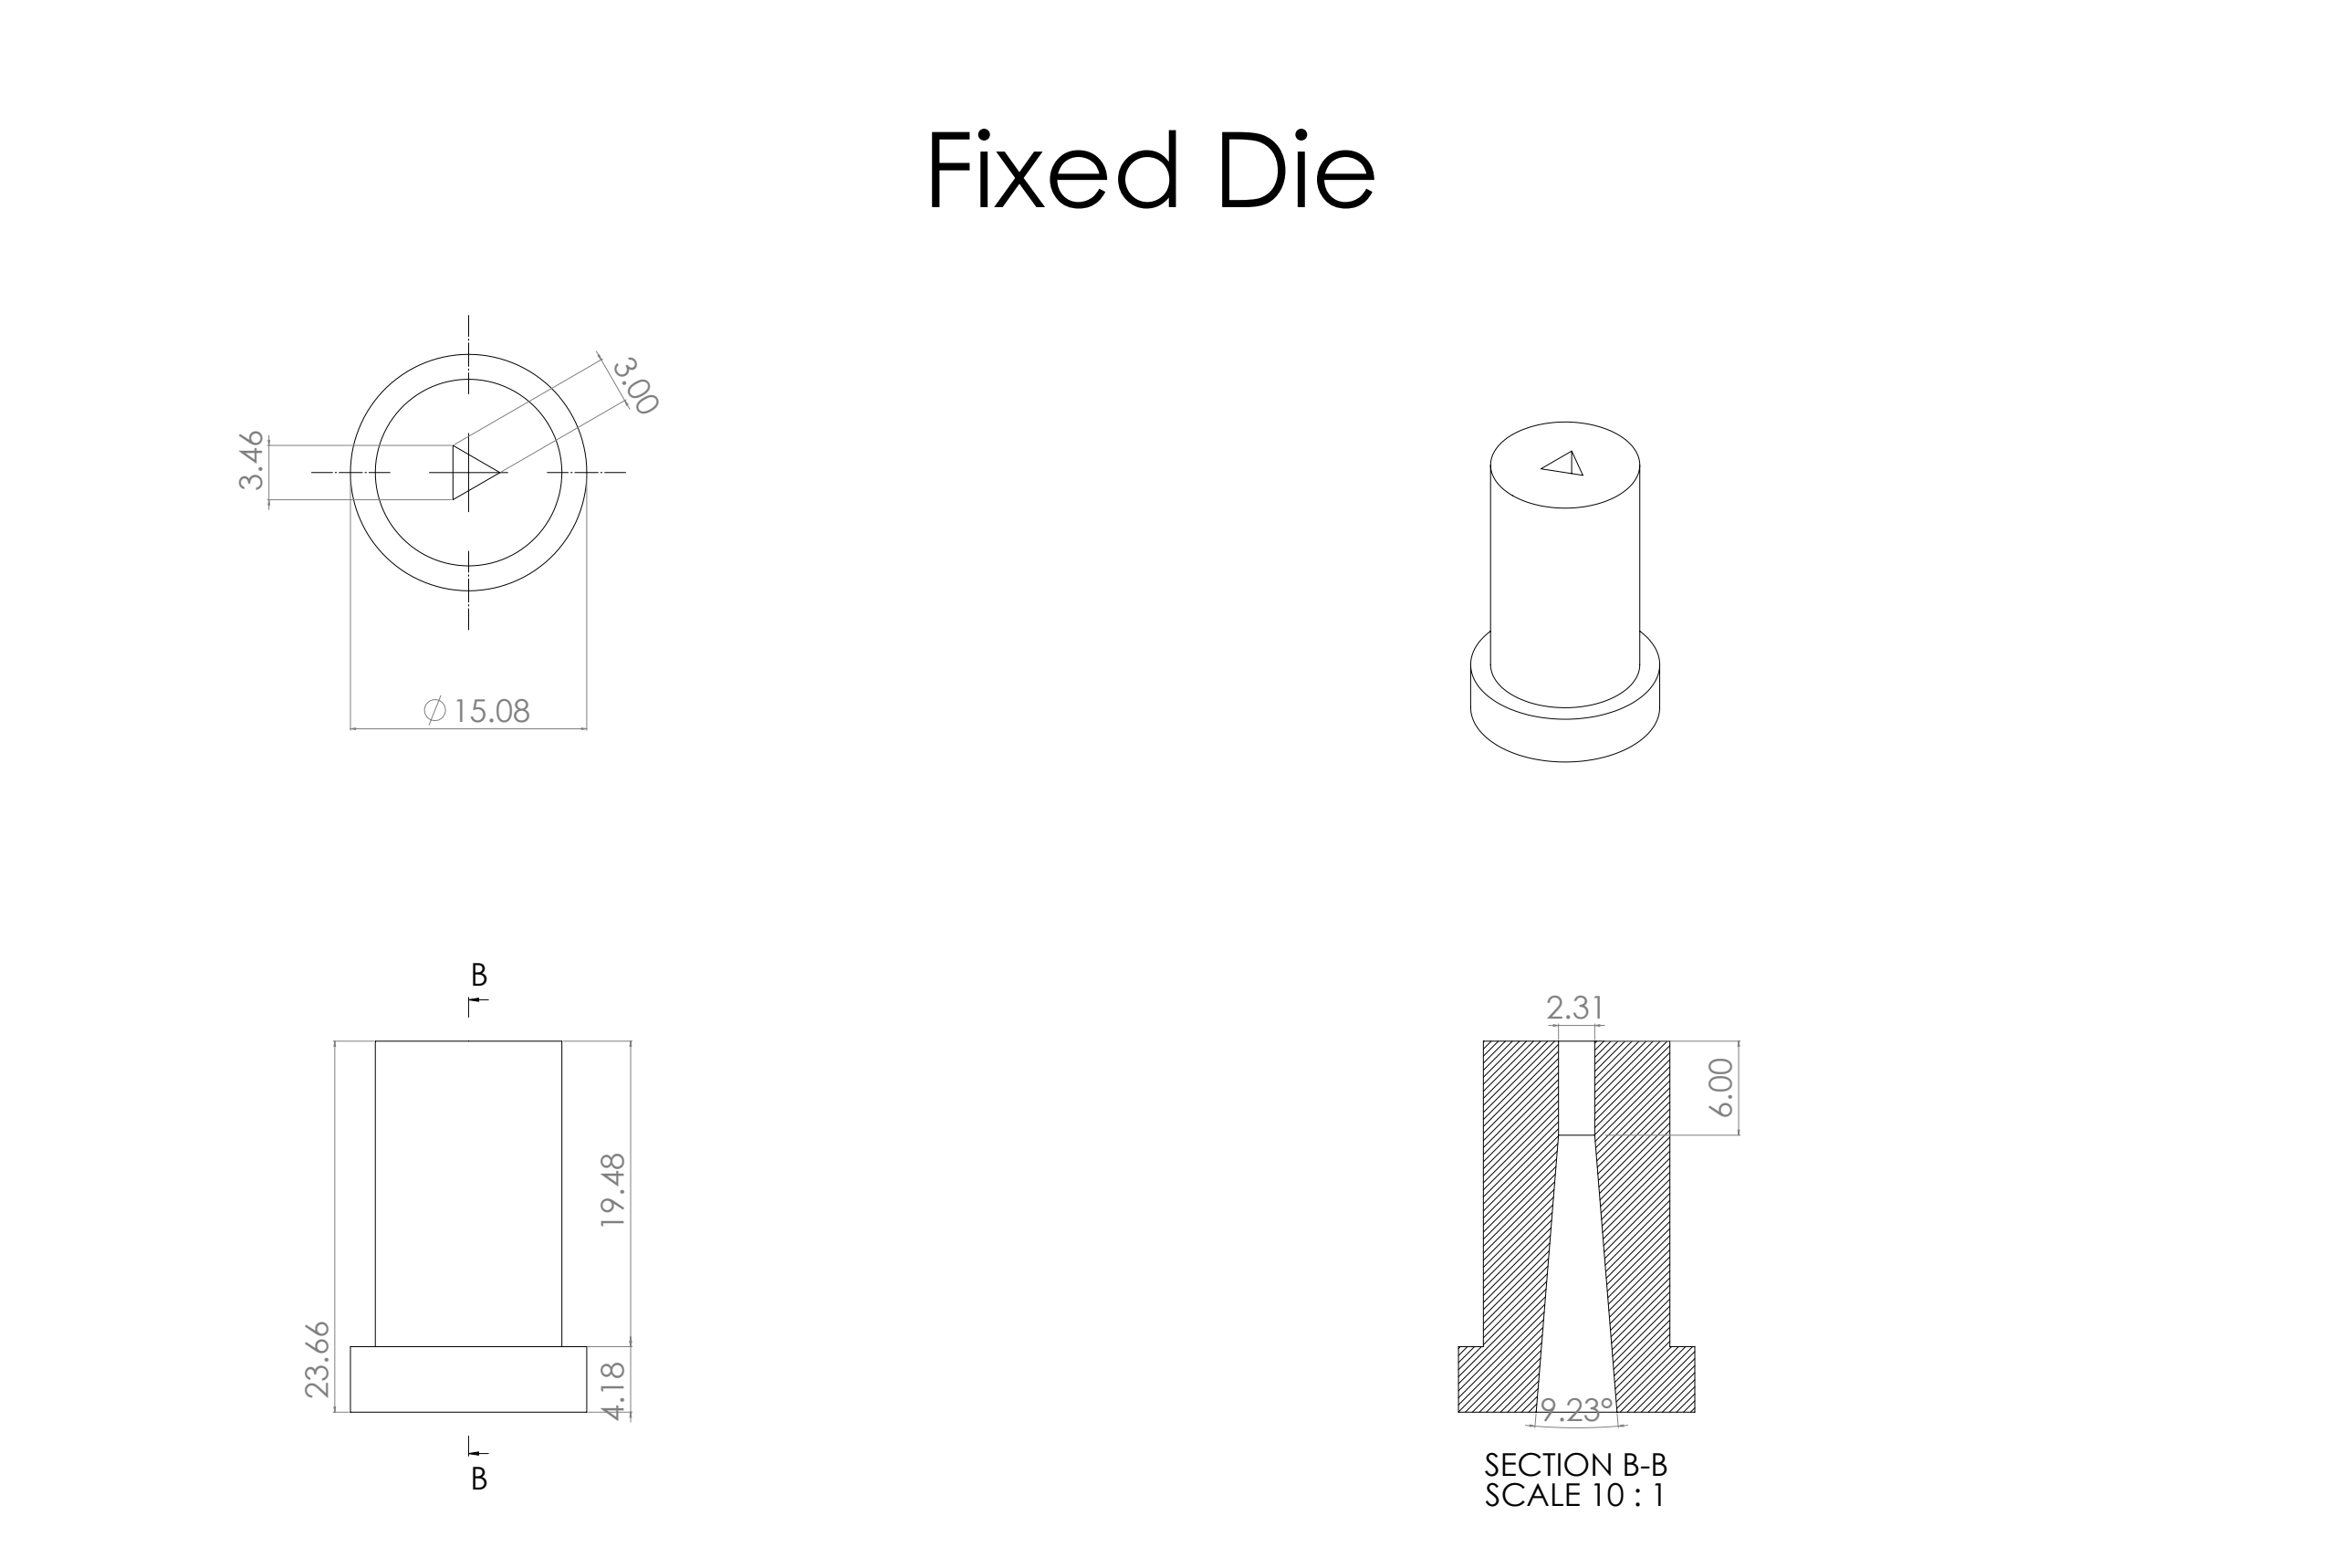
ISO-10303-21;
HEADER;
FILE_DESCRIPTION (('STEP AP214'),
    '1' );
FILE_NAME ('Fixed Die.step',
    '2026-10-24T22:54:28',
    ( '' ),
    ( '' ),
    'SwSTEP 2.0',
    'SolidWorks 2025',
    '' );
FILE_SCHEMA (( 'AUTOMOTIVE_DESIGN' ));
ENDSEC;

DATA;
#207=CARTESIAN_POINT ( 'NONE',  ( -71.92837670882106238, -36.87473357531881391, 0.000000000000000000 ) ) ;
#224=DIRECTION ( 'NONE',  ( 0.8660254037844378194, 0.000000000000000000, -0.5000000000000015543 ) ) ;
#393=VERTEX_POINT ( 'NONE', #4566 ) ;
#434=PLANE ( 'NONE',  #17404 ) ;
#625=EDGE_LOOP ( 'NONE', ( #4883, #27978 ) ) ;
#665=LINE ( 'NONE', #13201, #39699 ) ;
#902=LINE ( 'NONE', #25603, #35773 ) ;
#1067=( LENGTH_UNIT ( ) NAMED_UNIT ( * ) SI_UNIT ( .MILLI., .METRE. ) );
#1090=CARTESIAN_POINT ( 'NONE',  ( -70.92837670882107659, -56.35932253828836025, -7.538952224936807056 ) ) ;
#1093=EDGE_LOOP ( 'NONE', ( #23116, #22958, #9931 ) ) ;
#1109=EDGE_LOOP ( 'NONE', ( #22255, #22599 ) ) ;
#1161=EDGE_CURVE ( 'NONE', #12672, #5311, #17051, .T. ) ;
#1597=EDGE_CURVE ( 'NONE', #40141, #14437, #22702, .T. ) ;
#1683=CARTESIAN_POINT ( 'NONE',  ( -71.89960098016555889, -42.46322148352267334, 1.682209783512720325 ) ) ;
#1749=CARTESIAN_POINT ( 'NONE',  ( -70.92837670882107659, -36.87473357531881391, 5.950000000000010836 ) ) ;
#2203=DIRECTION ( 'NONE',  ( 0.000000000000000000, 1.000000000000000000, 0.000000000000000000 ) ) ;
#2209=DIRECTION ( 'NONE',  ( 0.000000000000000000, 0.000000000000000000, 1.000000000000000000 ) ) ;
#2300=AXIS2_PLACEMENT_3D ( 'NONE', #39101, #26169, #4151 ) ;
#2364=LINE ( 'NONE', #33652, #10169 ) ;
#2727=CARTESIAN_POINT ( 'NONE',  ( -64.15669616364040451, -60.53509472482660669, 1.328953532546354177 ) ) ;
#2806=DIRECTION ( 'NONE',  ( 0.000000000000000000, 1.000000000000000000, 0.000000000000000000 ) ) ;
#2845=PRODUCT_DEFINITION_CONTEXT ( 'detailed design', #4008, 'design' ) ;
#2876=PLANE ( 'NONE',  #36603 ) ;
#2926=DIRECTION ( 'NONE',  ( 0.000000000000000000, 0.000000000000000000, -1.000000000000000000 ) ) ;
#2936=VECTOR ( 'NONE', #14406, 1000.000000000000000 ) ;
#2937=VERTEX_POINT ( 'NONE', #1749 ) ;
#3000=CIRCLE ( 'NONE', #2300, 7.538952224936807056 ) ;
#3131=ORIENTED_EDGE ( 'NONE', *, *, #5528, .T. ) ;
#3396=DIRECTION ( 'NONE',  ( -0.000000000000000000, -1.000000000000000000, -0.000000000000000000 ) ) ;
#3415=LINE ( 'NONE', #15927, #25846 ) ;
#3420=FACE_OUTER_BOUND ( 'NONE', #15790, .T. ) ;
#3469=CARTESIAN_POINT ( 'NONE',  ( -70.92837670882107659, -56.35932253828836025, 0.000000000000000000 ) ) ;
#3553=DIRECTION ( 'NONE',  ( 1.000000000000000000, 0.000000000000000000, 0.000000000000000000 ) ) ;
#3613=EDGE_LOOP ( 'NONE', ( #15107, #25975, #24061, #17576 ) ) ;
#3750=( GEOMETRIC_REPRESENTATION_CONTEXT ( 3 ) GLOBAL_UNCERTAINTY_ASSIGNED_CONTEXT ( ( #25460 ) ) GLOBAL_UNIT_ASSIGNED_CONTEXT ( ( #39616, #24183, #17995 ) ) REPRESENTATION_CONTEXT ( 'NONE', 'WORKASPACE' ) );
#3827=CARTESIAN_POINT ( 'NONE',  ( -70.92837670882107659, -36.87473357531881391, 0.000000000000000000 ) ) ;
#3963=CARTESIAN_POINT ( 'NONE',  ( -71.92837670882106238, -42.87473357531881391, -1.732050807568860318 ) ) ;
#4008=APPLICATION_CONTEXT ( 'automotive_design' ) ;
#4151=DIRECTION ( 'NONE',  ( 0.000000000000000000, 0.000000000000000000, -1.000000000000000000 ) ) ;
#4259=DIRECTION ( 'NONE',  ( 0.000000000000000000, 0.000000000000000000, -1.000000000000000000 ) ) ;
#4566=CARTESIAN_POINT ( 'NONE',  ( -70.92837670882107659, -60.53509472482660669, 7.538952224936807056 ) ) ;
#4749=CARTESIAN_POINT ( 'NONE',  ( -66.45851120290885206, -60.53509472482660669, -7.806255641895631925E-15 ) ) ;
#4780=VERTEX_POINT ( 'NONE', #9078 ) ;
#4883=ORIENTED_EDGE ( 'NONE', *, *, #31531, .F. ) ;
#5208=VERTEX_POINT ( 'NONE', #4749 ) ;
#5311=VERTEX_POINT ( 'NONE', #14408 ) ;
#5366=ORIENTED_EDGE ( 'NONE', *, *, #5820, .T. ) ;
#5526=CARTESIAN_POINT ( 'NONE',  ( -71.92837670882106238, -42.87473357531881391, -1.732050807568860318 ) ) ;
#5528=EDGE_CURVE ( 'NONE', #24744, #4780, #6786, .T. ) ;
#5754=VERTEX_POINT ( 'NONE', #7183 ) ;
#5820=EDGE_CURVE ( 'NONE', #5754, #35842, #23779, .T. ) ;
#5942=CARTESIAN_POINT ( 'NONE',  ( -70.42837670882107659, -36.87473357531881391, -0.8660254037844368202 ) ) ;
#6122=AXIS2_PLACEMENT_3D ( 'NONE', #20569, #33156, #7623 ) ;
#6322=ORIENTED_EDGE ( 'NONE', *, *, #1161, .F. ) ;
#6624=CARTESIAN_POINT ( 'NONE',  ( -71.92837670882106238, -36.87473357531881391, -1.732050807568860318 ) ) ;
#6666=EDGE_CURVE ( 'NONE', #2937, #18869, #36703, .T. ) ;
#6714=AXIS2_PLACEMENT_3D ( 'NONE', #38265, #38664, #32717 ) ;
#6786=LINE ( 'NONE', #207, #20487 ) ;
#7021=FACE_OUTER_BOUND ( 'NONE', #11884, .T. ) ;
#7183=CARTESIAN_POINT ( 'NONE',  ( -70.92837670882107659, -56.35932253828836025, 7.538952224936807056 ) ) ;
#7203=CARTESIAN_POINT ( 'NONE',  ( -70.92837670882107659, -60.53509472482660669, -7.538952224936807056 ) ) ;
#7316=PRODUCT_CONTEXT ( 'NONE', #8952, 'mechanical' ) ;
#7549=DIRECTION ( 'NONE',  ( 0.000000000000000000, 0.000000000000000000, -1.000000000000000000 ) ) ;
#7594=DIRECTION ( 'NONE',  ( 0.8660254037844378194, 0.000000000000000000, -0.5000000000000015543 ) ) ;
#7623=DIRECTION ( 'NONE',  ( 0.8660254037844378194, 0.000000000000000000, -0.5000000000000015543 ) ) ;
#7919=SHAPE_DEFINITION_REPRESENTATION ( #12565, #32460 ) ;
#7949=EDGE_CURVE ( 'NONE', #22149, #393, #24947, .T. ) ;
#7985=CYLINDRICAL_SURFACE ( 'NONE', #23972, 5.950000000000010836 ) ;
#8004=DIRECTION ( 'NONE',  ( -0.000000000000000000, -1.000000000000000000, -0.000000000000000000 ) ) ;
#8100=ORIENTED_EDGE ( 'NONE', *, *, #8860, .T. ) ;
#8103=DIRECTION ( 'NONE',  ( -0.000000000000000000, 1.000000000000000000, -0.000000000000000000 ) ) ;
#8110=ORIENTED_EDGE ( 'NONE', *, *, #25965, .T. ) ;
#8132=CARTESIAN_POINT ( 'NONE',  ( -71.92837670882106238, -42.87473357531881391, 1.732050807568877637 ) ) ;
#8190=AXIS2_PLACEMENT_3D ( 'NONE', #18545, #27616, #27209 ) ;
#8239=PRODUCT ( 'Fixed Die', 'Fixed Die', '', ( #7316 ) ) ;
#8244=LINE ( 'NONE', #2727, #8578 ) ;
#8344=DIRECTION ( 'NONE',  ( 0.000000000000000000, -0.000000000000000000, 1.000000000000000000 ) ) ;
#8361=EDGE_LOOP ( 'NONE', ( #33245, #39618, #23431, #8597 ) ) ;
#8539=CARTESIAN_POINT ( 'NONE',  ( -71.92837670882106238, -42.87473357531881391, 1.732050807568877637 ) ) ;
#8569=UNCERTAINTY_MEASURE_WITH_UNIT (LENGTH_MEASURE( 1.000000000000000082E-05 ), #1067, 'distance_accuracy_value', 'NONE');
#8578=VECTOR ( 'NONE', #15250, 1000.000000000000114 ) ;
#8597=ORIENTED_EDGE ( 'NONE', *, *, #24404, .F. ) ;
#8860=EDGE_CURVE ( 'NONE', #2937, #5311, #17859, .T. ) ;
#8948=DIRECTION ( 'NONE',  ( 0.000000000000000000, 0.000000000000000000, -1.000000000000000000 ) ) ;
#8952=APPLICATION_CONTEXT ( 'automotive_design' ) ;
#8971=AXIS2_PLACEMENT_3D ( 'NONE', #30800, #2806, #27681 ) ;
#9068=CARTESIAN_POINT ( 'NONE',  ( -68.92837670882107659, -42.87473357531881391, 0.000000000000000000 ) ) ;
#9078=CARTESIAN_POINT ( 'NONE',  ( -71.92837670882106238, -36.87473357531881391, 1.732050807568877637 ) ) ;
#9085=DIRECTION ( 'NONE',  ( -0.000000000000000000, -1.000000000000000000, -0.000000000000000000 ) ) ;
#9329=EDGE_LOOP ( 'NONE', ( #30157, #30991, #26917 ) ) ;
#9485=DIRECTION ( 'NONE',  ( 0.000000000000000000, 0.000000000000000000, 1.000000000000000000 ) ) ;
#9529=CIRCLE ( 'NONE', #39079, 5.950000000000010836 ) ;
#9571=FACE_BOUND ( 'NONE', #1093, .T. ) ;
#9887=FACE_OUTER_BOUND ( 'NONE', #33067, .T. ) ;
#9931=ORIENTED_EDGE ( 'NONE', *, *, #10183, .F. ) ;
#10141=DIRECTION ( 'NONE',  ( 0.06925283225918045515, 0.9903616414705930238, 0.1199494240409451351 ) ) ;
#10152=DIRECTION ( 'NONE',  ( 0.000000000000000000, 0.000000000000000000, -1.000000000000000000 ) ) ;
#10169=VECTOR ( 'NONE', #15091, 1000.000000000000114 ) ;
#10183=EDGE_CURVE ( 'NONE', #21412, #5208, #8244, .T. ) ;
#10234=DIRECTION ( 'NONE',  ( -0.000000000000000000, -1.000000000000000000, -0.000000000000000000 ) ) ;
#11063=ORIENTED_EDGE ( 'NONE', *, *, #36631, .T. ) ;
#11143=AXIS2_PLACEMENT_3D ( 'NONE', #3469, #22995, #4259 ) ;
#11295=PLANE ( 'NONE',  #6122 ) ;
#11801=ORIENTED_EDGE ( 'NONE', *, *, #1597, .F. ) ;
#11884=EDGE_LOOP ( 'NONE', ( #26290, #20183, #23152, #11801 ) ) ;
#12137=ORIENTED_EDGE ( 'NONE', *, *, #12369, .F. ) ;
#12246=DIRECTION ( 'NONE',  ( 0.000000000000000000, -1.000000000000000000, -0.000000000000000000 ) ) ;
#12369=EDGE_CURVE ( 'NONE', #28633, #31670, #2364, .T. ) ;
#12447=AXIS2_PLACEMENT_3D ( 'NONE', #33798, #24304, #2926 ) ;
#12478=VECTOR ( 'NONE', #26746, 1000.000000000000000 ) ;
#12565=PRODUCT_DEFINITION_SHAPE ( 'NONE', 'NONE',  #27315 ) ;
#12595=EDGE_CURVE ( 'NONE', #18869, #2937, #9529, .T. ) ;
#12657=PLANE ( 'NONE',  #30715 ) ;
#12672=VERTEX_POINT ( 'NONE', #39135 ) ;
#12682=SHAPE_REPRESENTATION_RELATIONSHIP ( 'NONE' , 'NONE' ,  #32460, #31867 ) ;
#13056=ADVANCED_FACE ( 'NONE', ( #30915 ), #434, .F. ) ;
#13093=( NAMED_UNIT ( * ) PLANE_ANGLE_UNIT ( ) SI_UNIT ( $, .RADIAN. ) );
#13201=CARTESIAN_POINT ( 'NONE',  ( -64.15669616364041872, -60.53509472482660669, -1.328953532546369276 ) ) ;
#13407=FACE_BOUND ( 'NONE', #1109, .T. ) ;
#13587=EDGE_CURVE ( 'NONE', #15847, #24744, #21594, .T. ) ;
#14273=EDGE_LOOP ( 'NONE', ( #15186, #5366, #11063, #14688 ) ) ;
#14366=DIRECTION ( 'NONE',  ( -0.000000000000000000, -1.000000000000000000, -0.000000000000000000 ) ) ;
#14406=DIRECTION ( 'NONE',  ( 0.000000000000000000, 0.000000000000000000, -1.000000000000000000 ) ) ;
#14408=CARTESIAN_POINT ( 'NONE',  ( -70.92837670882107659, -56.35932253828836025, 5.950000000000010836 ) ) ;
#14437=VERTEX_POINT ( 'NONE', #8132 ) ;
#14588=EDGE_CURVE ( 'NONE', #5754, #393, #18017, .T. ) ;
#14637=FACE_OUTER_BOUND ( 'NONE', #8361, .T. ) ;
#14662=DIRECTION ( 'NONE',  ( 0.000000000000000000, 0.000000000000000000, -1.000000000000000000 ) ) ;
#14688=ORIENTED_EDGE ( 'NONE', *, *, #22477, .F. ) ;
#14692=CARTESIAN_POINT ( 'NONE',  ( -68.92837670882107659, -42.87473357531881391, 0.000000000000000000 ) ) ;
#14716=DIRECTION ( 'NONE',  ( -0.000000000000000000, -1.000000000000000000, -0.000000000000000000 ) ) ;
#14961=CARTESIAN_POINT ( 'NONE',  ( -73.16330946177717465, -60.53509472482661380, 3.871017079619767376 ) ) ;
#14986=ORIENTED_EDGE ( 'NONE', *, *, #28741, .T. ) ;
#15091=DIRECTION ( 'NONE',  ( -0.8660254037844399289, 0.000000000000000000, -0.4999999999999977240 ) ) ;
#15107=ORIENTED_EDGE ( 'NONE', *, *, #30928, .T. ) ;
#15126=PLANE ( 'NONE',  #8971 ) ;
#15186=ORIENTED_EDGE ( 'NONE', *, *, #14588, .F. ) ;
#15223=ORIENTED_EDGE ( 'NONE', *, *, #13587, .T. ) ;
#15250=DIRECTION ( 'NONE',  ( 0.8660254037844399289, 0.000000000000000000, 0.4999999999999976685 ) ) ;
#15444=ORIENTED_EDGE ( 'NONE', *, *, #12595, .F. ) ;
#15510=VECTOR ( 'NONE', #27833, 1000.000000000000114 ) ;
#15608=DIRECTION ( 'NONE',  ( 0.000000000000000000, 0.000000000000000000, 1.000000000000000000 ) ) ;
#15636=ADVANCED_FACE ( 'NONE', ( #38836 ), #35775, .T. ) ;
#15670=ADVANCED_FACE ( 'NONE', ( #23604, #33503 ), #18022, .T. ) ;
#15737=ORIENTED_EDGE ( 'NONE', *, *, #22477, .T. ) ;
#15790=EDGE_LOOP ( 'NONE', ( #32669, #22324, #37632, #26866 ) ) ;
#15832=ORIENTED_EDGE ( 'NONE', *, *, #32968, .T. ) ;
#15847=VERTEX_POINT ( 'NONE', #40074 ) ;
#15861=DIRECTION ( 'NONE',  ( -0.8660254037844399289, 0.000000000000000000, -0.4999999999999977240 ) ) ;
#15927=CARTESIAN_POINT ( 'NONE',  ( -71.92837670882106238, -42.87473357531881391, 1.732050807568877637 ) ) ;
#16115=CARTESIAN_POINT ( 'NONE',  ( -70.92837670882107659, -36.87473357531881391, 0.000000000000000000 ) ) ;
#16212=MECHANICAL_DESIGN_GEOMETRIC_PRESENTATION_REPRESENTATION('',(#39862),#3750);
#16213=VECTOR ( 'NONE', #30275, 1000.000000000000000 ) ;
#16974=LINE ( 'NONE', #14692, #28770 ) ;
#17017=ORIENTED_EDGE ( 'NONE', *, *, #12595, .T. ) ;
#17051=CIRCLE ( 'NONE', #11143, 5.950000000000010836 ) ;
#17091=CARTESIAN_POINT ( 'NONE',  ( -70.92837670882107659, -60.53509472482660669, -7.538952224936807056 ) ) ;
#17193=CARTESIAN_POINT ( 'NONE',  ( -71.92837670882106238, -42.87473357531881391, -1.732050807568860318 ) ) ;
#17300=AXIS2_PLACEMENT_3D ( 'NONE', #29110, #31800, #10152 ) ;
#17386=DIRECTION ( 'NONE',  ( -0.000000000000000000, 1.000000000000000000, -0.000000000000000000 ) ) ;
#17404=AXIS2_PLACEMENT_3D ( 'NONE', #37665, #18954, #224 ) ;
#17484=LINE ( 'NONE', #17091, #16213 ) ;
#17576=ORIENTED_EDGE ( 'NONE', *, *, #31764, .T. ) ;
#17612=CARTESIAN_POINT ( 'NONE',  ( -71.92837670882106238, -42.87473357531881391, -1.732050807568860318 ) ) ;
#17763=CARTESIAN_POINT ( 'NONE',  ( -73.16330946177717465, -60.53509472482659959, -3.871017079619738510 ) ) ;
#17820=LINE ( 'NONE', #17612, #26678 ) ;
#17859=LINE ( 'NONE', #30440, #12478 ) ;
#17995=( NAMED_UNIT ( * ) SI_UNIT ( $, .STERADIAN. ) SOLID_ANGLE_UNIT ( ) );
#18017=LINE ( 'NONE', #36559, #24725 ) ;
#18022=PLANE ( 'NONE',  #20626 ) ;
#18066=VECTOR ( 'NONE', #31067, 1000.000000000000114 ) ;
#18376=DIRECTION ( 'NONE',  ( -0.000000000000000000, 1.000000000000000000, -0.000000000000000000 ) ) ;
#18545=CARTESIAN_POINT ( 'NONE',  ( -68.92837670882107659, -42.87473357531881391, 0.000000000000000000 ) ) ;
#18660=AXIS2_PLACEMENT_3D ( 'NONE', #28786, #10234, #7549 ) ;
#18787=LINE ( 'NONE', #31365, #39256 ) ;
#18869=VERTEX_POINT ( 'NONE', #19058 ) ;
#18954=DIRECTION ( 'NONE',  ( 0.5000000000000015543, 0.000000000000000000, 0.8660254037844378194 ) ) ;
#19058=CARTESIAN_POINT ( 'NONE',  ( -70.92837670882107659, -36.87473357531881391, -5.950000000000010836 ) ) ;
#19589=PLANE ( 'NONE',  #33092 ) ;
#19592=VECTOR ( 'NONE', #17386, 1000.000000000000000 ) ;
#19700=LINE ( 'NONE', #8539, #19592 ) ;
#20177=DIRECTION ( 'NONE',  ( -0.9975640502598243087, 0.06975647374412531632, 0.000000000000000000 ) ) ;
#20183=ORIENTED_EDGE ( 'NONE', *, *, #24404, .T. ) ;
#20210=ADVANCED_FACE ( 'NONE', ( #36707 ), #20645, .T. ) ;
#20341=CARTESIAN_POINT ( 'NONE',  ( -70.42837670882107659, -36.87473357531881391, 0.8660254037844411501 ) ) ;
#20487=VECTOR ( 'NONE', #22033, 1000.000000000000000 ) ;
#20541=CARTESIAN_POINT ( 'NONE',  ( -70.92837670882107659, -60.53509472482660669, 0.000000000000000000 ) ) ;
#20569=CARTESIAN_POINT ( 'NONE',  ( -71.92837670882106238, -42.87473357531881391, 1.732050807568877637 ) ) ;
#20576=ORIENTED_EDGE ( 'NONE', *, *, #25965, .F. ) ;
#20617=ADVANCED_FACE ( 'NONE', ( #39074 ), #7985, .T. ) ;
#20626=AXIS2_PLACEMENT_3D ( 'NONE', #36168, #2203, #8344 ) ;
#20645=CYLINDRICAL_SURFACE ( 'NONE', #34514, 7.538952224936807056 ) ;
#20898=CIRCLE ( 'NONE', #35390, 7.538952224936807056 ) ;
#21412=VERTEX_POINT ( 'NONE', #17763 ) ;
#21594=LINE ( 'NONE', #5942, #18066 ) ;
#21733=FACE_OUTER_BOUND ( 'NONE', #32261, .T. ) ;
#21889=ORIENTED_EDGE ( 'NONE', *, *, #1597, .T. ) ;
#21909=ADVANCED_FACE ( 'NONE', ( #9887 ), #37271, .F. ) ;
#22033=DIRECTION ( 'NONE',  ( 0.000000000000000000, -0.000000000000000000, 1.000000000000000000 ) ) ;
#22075=LINE ( 'NONE', #25149, #40308 ) ;
#22128=ORIENTED_EDGE ( 'NONE', *, *, #7949, .T. ) ;
#22149=VERTEX_POINT ( 'NONE', #7203 ) ;
#22255=ORIENTED_EDGE ( 'NONE', *, *, #1161, .T. ) ;
#22276=ADVANCED_FACE ( 'NONE', ( #14637 ), #34238, .F. ) ;
#22324=ORIENTED_EDGE ( 'NONE', *, *, #14588, .T. ) ;
#22400=DIRECTION ( 'NONE',  ( 0.000000000000000000, 0.000000000000000000, -1.000000000000000000 ) ) ;
#22477=EDGE_CURVE ( 'NONE', #393, #22149, #3000, .T. ) ;
#22599=ORIENTED_EDGE ( 'NONE', *, *, #27281, .T. ) ;
#22702=LINE ( 'NONE', #1683, #22993 ) ;
#22958=ORIENTED_EDGE ( 'NONE', *, *, #32968, .F. ) ;
#22993=VECTOR ( 'NONE', #33172, 999.9999999999998863 ) ;
#22995=DIRECTION ( 'NONE',  ( -0.000000000000000000, -1.000000000000000000, -0.000000000000000000 ) ) ;
#23088=DIRECTION ( 'NONE',  ( -0.8660254037844377084, 0.000000000000000000, 0.5000000000000015543 ) ) ;
#23116=ORIENTED_EDGE ( 'NONE', *, *, #23514, .F. ) ;
#23144=DIRECTION ( 'NONE',  ( -0.000000000000000000, -1.000000000000000000, -0.000000000000000000 ) ) ;
#23152=ORIENTED_EDGE ( 'NONE', *, *, #35047, .T. ) ;
#23167=CIRCLE ( 'NONE', #32379, 5.950000000000010836 ) ;
#23431=ORIENTED_EDGE ( 'NONE', *, *, #12369, .T. ) ;
#23514=EDGE_CURVE ( 'NONE', #40141, #21412, #33163, .T. ) ;
#23604=FACE_BOUND ( 'NONE', #9329, .T. ) ;
#23626=ORIENTED_EDGE ( 'NONE', *, *, #38478, .T. ) ;
#23779=CIRCLE ( 'NONE', #6714, 7.538952224936807056 ) ;
#23972=AXIS2_PLACEMENT_3D ( 'NONE', #20541, #14366, #26934 ) ;
#24061=ORIENTED_EDGE ( 'NONE', *, *, #25439, .F. ) ;
#24183=( NAMED_UNIT ( * ) PLANE_ANGLE_UNIT ( ) SI_UNIT ( $, .RADIAN. ) );
#24234=CLOSED_SHELL ( 'NONE', ( #32471, #20617, #28192, #15670, #15636, #34100, #20210, #13056, #37278, #21909, #26152, #22276, #26184 ) ) ;
#24304=DIRECTION ( 'NONE',  ( -0.000000000000000000, -1.000000000000000000, -0.000000000000000000 ) ) ;
#24404=EDGE_CURVE ( 'NONE', #21412, #31670, #902, .T. ) ;
#24617=AXIS2_PLACEMENT_3D ( 'NONE', #9068, #34223, #15861 ) ;
#24670=DIRECTION ( 'NONE',  ( -1.000000000000000000, 0.000000000000000000, 0.000000000000000000 ) ) ;
#24725=VECTOR ( 'NONE', #14716, 1000.000000000000000 ) ;
#24744=VERTEX_POINT ( 'NONE', #6624 ) ;
#24947=CIRCLE ( 'NONE', #12447, 7.538952224936807056 ) ;
#24969=CARTESIAN_POINT ( 'NONE',  ( -68.98592816613208356, -42.46322148352267334, -2.168404344971008868E-16 ) ) ;
#24996=ORIENTED_EDGE ( 'NONE', *, *, #35047, .F. ) ;
#25149=CARTESIAN_POINT ( 'NONE',  ( -70.92837670882107659, -60.53509472482660669, -5.950000000000010836 ) ) ;
#25374=LINE ( 'NONE', #24969, #15510 ) ;
#25439=EDGE_CURVE ( 'NONE', #14437, #28633, #3415, .T. ) ;
#25460=UNCERTAINTY_MEASURE_WITH_UNIT (LENGTH_MEASURE( 1.000000000000000082E-05 ), #39616, 'distance_accuracy_value', 'NONE');
#25507=ORIENTED_EDGE ( 'NONE', *, *, #8860, .F. ) ;
#25603=CARTESIAN_POINT ( 'NONE',  ( -71.89960098016555889, -42.46322148352267334, -1.682209783512703227 ) ) ;
#25752=EDGE_LOOP ( 'NONE', ( #17017, #8100, #6322, #20576 ) ) ;
#25846=VECTOR ( 'NONE', #37541, 1000.000000000000000 ) ;
#25965=EDGE_CURVE ( 'NONE', #18869, #12672, #22075, .T. ) ;
#25975=ORIENTED_EDGE ( 'NONE', *, *, #38478, .F. ) ;
#26121=VECTOR ( 'NONE', #7594, 1000.000000000000000 ) ;
#26152=ADVANCED_FACE ( 'NONE', ( #7021 ), #19589, .F. ) ;
#26169=DIRECTION ( 'NONE',  ( -0.000000000000000000, -1.000000000000000000, -0.000000000000000000 ) ) ;
#26184=ADVANCED_FACE ( 'NONE', ( #36236 ), #11295, .F. ) ;
#26288=EDGE_LOOP ( 'NONE', ( #3131, #28796, #24996, #14986 ) ) ;
#26290=ORIENTED_EDGE ( 'NONE', *, *, #23514, .T. ) ;
#26678=VECTOR ( 'NONE', #2209, 1000.000000000000000 ) ;
#26746=DIRECTION ( 'NONE',  ( -0.000000000000000000, -1.000000000000000000, -0.000000000000000000 ) ) ;
#26866=ORIENTED_EDGE ( 'NONE', *, *, #36631, .F. ) ;
#26917=ORIENTED_EDGE ( 'NONE', *, *, #13587, .F. ) ;
#26934=DIRECTION ( 'NONE',  ( 0.000000000000000000, 0.000000000000000000, -1.000000000000000000 ) ) ;
#27209=DIRECTION ( 'NONE',  ( -0.8660254037844399289, 0.000000000000000000, -0.4999999999999976685 ) ) ;
#27281=EDGE_CURVE ( 'NONE', #5311, #12672, #23167, .T. ) ;
#27315=PRODUCT_DEFINITION ( 'UNKNOWN', '', #36025, #2845 ) ;
#27429=( GEOMETRIC_REPRESENTATION_CONTEXT ( 3 ) GLOBAL_UNCERTAINTY_ASSIGNED_CONTEXT ( ( #8569 ) ) GLOBAL_UNIT_ASSIGNED_CONTEXT ( ( #1067, #13093, #35148 ) ) REPRESENTATION_CONTEXT ( 'NONE', 'WORKASPACE' ) );
#27462=ORIENTED_EDGE ( 'NONE', *, *, #25439, .T. ) ;
#27616=DIRECTION ( 'NONE',  ( 0.4987820251299098784, 0.06975647374412531632, -0.8639158094271057742 ) ) ;
#27681=DIRECTION ( 'NONE',  ( 0.000000000000000000, -0.000000000000000000, 1.000000000000000000 ) ) ;
#27833=DIRECTION ( 'NONE',  ( -0.1385056645183609658, 0.9903616414705929127, 3.027401012299304875E-16 ) ) ;
#27890=CARTESIAN_POINT ( 'NONE',  ( -63.38942448388426243, -60.53509472482660669, 0.000000000000000000 ) ) ;
#27978=ORIENTED_EDGE ( 'NONE', *, *, #5820, .F. ) ;
#28192=ADVANCED_FACE ( 'NONE', ( #9571, #21733 ), #12657, .T. ) ;
#28633=VERTEX_POINT ( 'NONE', #36511 ) ;
#28741=EDGE_CURVE ( 'NONE', #31670, #24744, #18787, .T. ) ;
#28770=VECTOR ( 'NONE', #8103, 1000.000000000000000 ) ;
#28786=CARTESIAN_POINT ( 'NONE',  ( -70.92837670882107659, -60.53509472482660669, 0.000000000000000000 ) ) ;
#28796=ORIENTED_EDGE ( 'NONE', *, *, #31764, .F. ) ;
#29110=CARTESIAN_POINT ( 'NONE',  ( -70.92837670882107659, -60.53509472482660669, 0.000000000000000000 ) ) ;
#29322=DIRECTION ( 'NONE',  ( 0.000000000000000000, 0.000000000000000000, 1.000000000000000000 ) ) ;
#29452=EDGE_LOOP ( 'NONE', ( #15444, #39629 ) ) ;
#30069=CARTESIAN_POINT ( 'NONE',  ( -73.16330946177717465, -60.53509472482660669, 0.000000000000000000 ) ) ;
#30157=ORIENTED_EDGE ( 'NONE', *, *, #30928, .F. ) ;
#30275=DIRECTION ( 'NONE',  ( -0.000000000000000000, -1.000000000000000000, -0.000000000000000000 ) ) ;
#30440=CARTESIAN_POINT ( 'NONE',  ( -70.92837670882107659, -60.53509472482660669, 5.950000000000010836 ) ) ;
#30715=AXIS2_PLACEMENT_3D ( 'NONE', #27890, #12246, #8948 ) ;
#30744=AXIS2_PLACEMENT_3D ( 'NONE', #35448, #9485, #3553 ) ;
#30800=CARTESIAN_POINT ( 'NONE',  ( -64.97837670882105954, -56.35932253828836025, 0.000000000000000000 ) ) ;
#30852=ORIENTED_EDGE ( 'NONE', *, *, #27281, .F. ) ;
#30915=FACE_OUTER_BOUND ( 'NONE', #3613, .T. ) ;
#30928=EDGE_CURVE ( 'NONE', #4780, #15847, #35424, .T. ) ;
#30991=ORIENTED_EDGE ( 'NONE', *, *, #5528, .F. ) ;
#31059=ORIENTED_EDGE ( 'NONE', *, *, #6666, .T. ) ;
#31067=DIRECTION ( 'NONE',  ( -0.8660254037844399289, 0.000000000000000000, -0.4999999999999977240 ) ) ;
#31167=DIRECTION ( 'NONE',  ( 0.000000000000000000, 0.000000000000000000, 1.000000000000000000 ) ) ;
#31365=CARTESIAN_POINT ( 'NONE',  ( -71.92837670882106238, -42.87473357531881391, -1.732050807568860318 ) ) ;
#31531=EDGE_CURVE ( 'NONE', #35842, #5754, #20898, .T. ) ;
#31670=VERTEX_POINT ( 'NONE', #17193 ) ;
#31689=ORIENTED_EDGE ( 'NONE', *, *, #36400, .F. ) ;
#31764=EDGE_CURVE ( 'NONE', #14437, #4780, #19700, .T. ) ;
#31800=DIRECTION ( 'NONE',  ( -0.000000000000000000, -1.000000000000000000, -0.000000000000000000 ) ) ;
#31867=ADVANCED_BREP_SHAPE_REPRESENTATION ( '', ( #39399, #30744 ), #27429 ) ;
#32261=EDGE_LOOP ( 'NONE', ( #22128, #15737 ) ) ;
#32379=AXIS2_PLACEMENT_3D ( 'NONE', #36034, #8004, #39499 ) ;
#32460=SHAPE_REPRESENTATION ( 'Fixed Die', ( #30744 ), #27429 ) ;
#32471=ADVANCED_FACE ( 'NONE', ( #3420 ), #38155, .T. ) ;
#32669=ORIENTED_EDGE ( 'NONE', *, *, #31531, .T. ) ;
#32717=DIRECTION ( 'NONE',  ( 0.000000000000000000, 0.000000000000000000, -1.000000000000000000 ) ) ;
#32968=EDGE_CURVE ( 'NONE', #5208, #40141, #665, .T. ) ;
#33067=EDGE_LOOP ( 'NONE', ( #15223, #34904, #12137, #23626 ) ) ;
#33092=AXIS2_PLACEMENT_3D ( 'NONE', #3963, #20177, #36437 ) ;
#33156=DIRECTION ( 'NONE',  ( 0.4987820251299136531, 0.06975647374412531632, 0.8639158094271034427 ) ) ;
#33163=LINE ( 'NONE', #30069, #2936 ) ;
#33172=DIRECTION ( 'NONE',  ( 0.06925283225918045515, 0.9903616414705930238, -0.1199494240409457457 ) ) ;
#33245=ORIENTED_EDGE ( 'NONE', *, *, #10183, .T. ) ;
#33503=FACE_OUTER_BOUND ( 'NONE', #29452, .T. ) ;
#33644=DIRECTION ( 'NONE',  ( -0.000000000000000000, -1.000000000000000000, -0.000000000000000000 ) ) ;
#33652=CARTESIAN_POINT ( 'NONE',  ( -68.92837670882107659, -42.87473357531881391, 0.000000000000000000 ) ) ;
#33798=CARTESIAN_POINT ( 'NONE',  ( -70.92837670882107659, -60.53509472482660669, 0.000000000000000000 ) ) ;
#34100=ADVANCED_FACE ( 'NONE', ( #13407, #35463 ), #15126, .T. ) ;
#34223=DIRECTION ( 'NONE',  ( 0.4999999999999977240, 0.000000000000000000, -0.8660254037844399289 ) ) ;
#34238=PLANE ( 'NONE',  #8190 ) ;
#34361=DIRECTION ( 'NONE',  ( -0.000000000000000000, -1.000000000000000000, -0.000000000000000000 ) ) ;
#34514=AXIS2_PLACEMENT_3D ( 'NONE', #37112, #33644, #14662 ) ;
#34904=ORIENTED_EDGE ( 'NONE', *, *, #28741, .F. ) ;
#35047=EDGE_CURVE ( 'NONE', #31670, #14437, #17820, .T. ) ;
#35148=( NAMED_UNIT ( * ) SI_UNIT ( $, .STERADIAN. ) SOLID_ANGLE_UNIT ( ) );
#35300=EDGE_LOOP ( 'NONE', ( #15832, #21889, #27462, #31689 ) ) ;
#35390=AXIS2_PLACEMENT_3D ( 'NONE', #37607, #34361, #22400 ) ;
#35424=LINE ( 'NONE', #20341, #26121 ) ;
#35448=CARTESIAN_POINT ( 'NONE',  ( 0.000000000000000000, 0.000000000000000000, 0.000000000000000000 ) ) ;
#35463=FACE_OUTER_BOUND ( 'NONE', #625, .T. ) ;
#35773=VECTOR ( 'NONE', #10141, 1000.000000000000000 ) ;
#35775=CYLINDRICAL_SURFACE ( 'NONE', #18660, 5.950000000000010836 ) ;
#35842=VERTEX_POINT ( 'NONE', #1090 ) ;
#36025=PRODUCT_DEFINITION_FORMATION_WITH_SPECIFIED_SOURCE ( 'ANY', '', #8239, .NOT_KNOWN. ) ;
#36034=CARTESIAN_POINT ( 'NONE',  ( -70.92837670882107659, -56.35932253828836025, 0.000000000000000000 ) ) ;
#36168=CARTESIAN_POINT ( 'NONE',  ( -70.92837670882107659, -36.87473357531881391, 0.000000000000000000 ) ) ;
#36236=FACE_OUTER_BOUND ( 'NONE', #35300, .T. ) ;
#36400=EDGE_CURVE ( 'NONE', #5208, #28633, #25374, .T. ) ;
#36437=DIRECTION ( 'NONE',  ( -0.06975647374412530244, -0.9975640502598241977, 0.000000000000000000 ) ) ;
#36511=CARTESIAN_POINT ( 'NONE',  ( -68.92837670882107659, -42.87473357531881391, 0.000000000000000000 ) ) ;
#36559=CARTESIAN_POINT ( 'NONE',  ( -70.92837670882107659, -60.53509472482660669, 7.538952224936807056 ) ) ;
#36603=AXIS2_PLACEMENT_3D ( 'NONE', #5526, #24670, #15608 ) ;
#36631=EDGE_CURVE ( 'NONE', #35842, #22149, #17484, .T. ) ;
#36703=CIRCLE ( 'NONE', #39997, 5.950000000000010836 ) ;
#36707=FACE_OUTER_BOUND ( 'NONE', #14273, .T. ) ;
#37112=CARTESIAN_POINT ( 'NONE',  ( -70.92837670882107659, -60.53509472482660669, 0.000000000000000000 ) ) ;
#37271=PLANE ( 'NONE',  #24617 ) ;
#37278=ADVANCED_FACE ( 'NONE', ( #37422 ), #2876, .F. ) ;
#37422=FACE_OUTER_BOUND ( 'NONE', #26288, .T. ) ;
#37541=DIRECTION ( 'NONE',  ( 0.8660254037844378194, 0.000000000000000000, -0.5000000000000015543 ) ) ;
#37607=CARTESIAN_POINT ( 'NONE',  ( -70.92837670882107659, -56.35932253828836025, 0.000000000000000000 ) ) ;
#37632=ORIENTED_EDGE ( 'NONE', *, *, #7949, .F. ) ;
#37665=CARTESIAN_POINT ( 'NONE',  ( -71.92837670882106238, -42.87473357531881391, 1.732050807568877637 ) ) ;
#38155=CYLINDRICAL_SURFACE ( 'NONE', #17300, 7.538952224936807056 ) ;
#38265=CARTESIAN_POINT ( 'NONE',  ( -70.92837670882107659, -56.35932253828836025, 0.000000000000000000 ) ) ;
#38478=EDGE_CURVE ( 'NONE', #28633, #15847, #16974, .T. ) ;
#38664=DIRECTION ( 'NONE',  ( -0.000000000000000000, -1.000000000000000000, -0.000000000000000000 ) ) ;
#38836=FACE_OUTER_BOUND ( 'NONE', #39667, .T. ) ;
#39074=FACE_OUTER_BOUND ( 'NONE', #25752, .T. ) ;
#39079=AXIS2_PLACEMENT_3D ( 'NONE', #16115, #3396, #31167 ) ;
#39101=CARTESIAN_POINT ( 'NONE',  ( -70.92837670882107659, -60.53509472482660669, 0.000000000000000000 ) ) ;
#39135=CARTESIAN_POINT ( 'NONE',  ( -70.92837670882107659, -56.35932253828836025, -5.950000000000010836 ) ) ;
#39256=VECTOR ( 'NONE', #18376, 1000.000000000000000 ) ;
#39399=MANIFOLD_SOLID_BREP ( 'Move Face3', #24234 ) ;
#39499=DIRECTION ( 'NONE',  ( 0.000000000000000000, 0.000000000000000000, -1.000000000000000000 ) ) ;
#39616=( LENGTH_UNIT ( ) NAMED_UNIT ( * ) SI_UNIT ( .MILLI., .METRE. ) );
#39618=ORIENTED_EDGE ( 'NONE', *, *, #36400, .T. ) ;
#39629=ORIENTED_EDGE ( 'NONE', *, *, #6666, .F. ) ;
#39667=EDGE_LOOP ( 'NONE', ( #25507, #31059, #8110, #30852 ) ) ;
#39699=VECTOR ( 'NONE', #23088, 1000.000000000000227 ) ;
#39862=STYLED_ITEM('',(#40773),#39399);
#39997=AXIS2_PLACEMENT_3D ( 'NONE', #3827, #23144, #29322 ) ;
#40074=CARTESIAN_POINT ( 'NONE',  ( -68.92837670882107659, -36.87473357531881391, 0.000000000000000000 ) ) ;
#40141=VERTEX_POINT ( 'NONE', #14961 ) ;
#40308=VECTOR ( 'NONE', #9085, 1000.000000000000000 ) ;
#40767=COLOUR_RGB('Off White',0.89,0.88,0.83);
#40768=FILL_AREA_STYLE_COLOUR('',#40767);
#40769=FILL_AREA_STYLE('',(#40768));
#40770=SURFACE_STYLE_FILL_AREA(#40769);
#40771=SURFACE_SIDE_STYLE('',(#40770));
#40772=SURFACE_STYLE_USAGE(.BOTH.,#40771);
#40773=PRESENTATION_STYLE_ASSIGNMENT((#40772));
ENDSEC;
END-ISO-10303-21;
